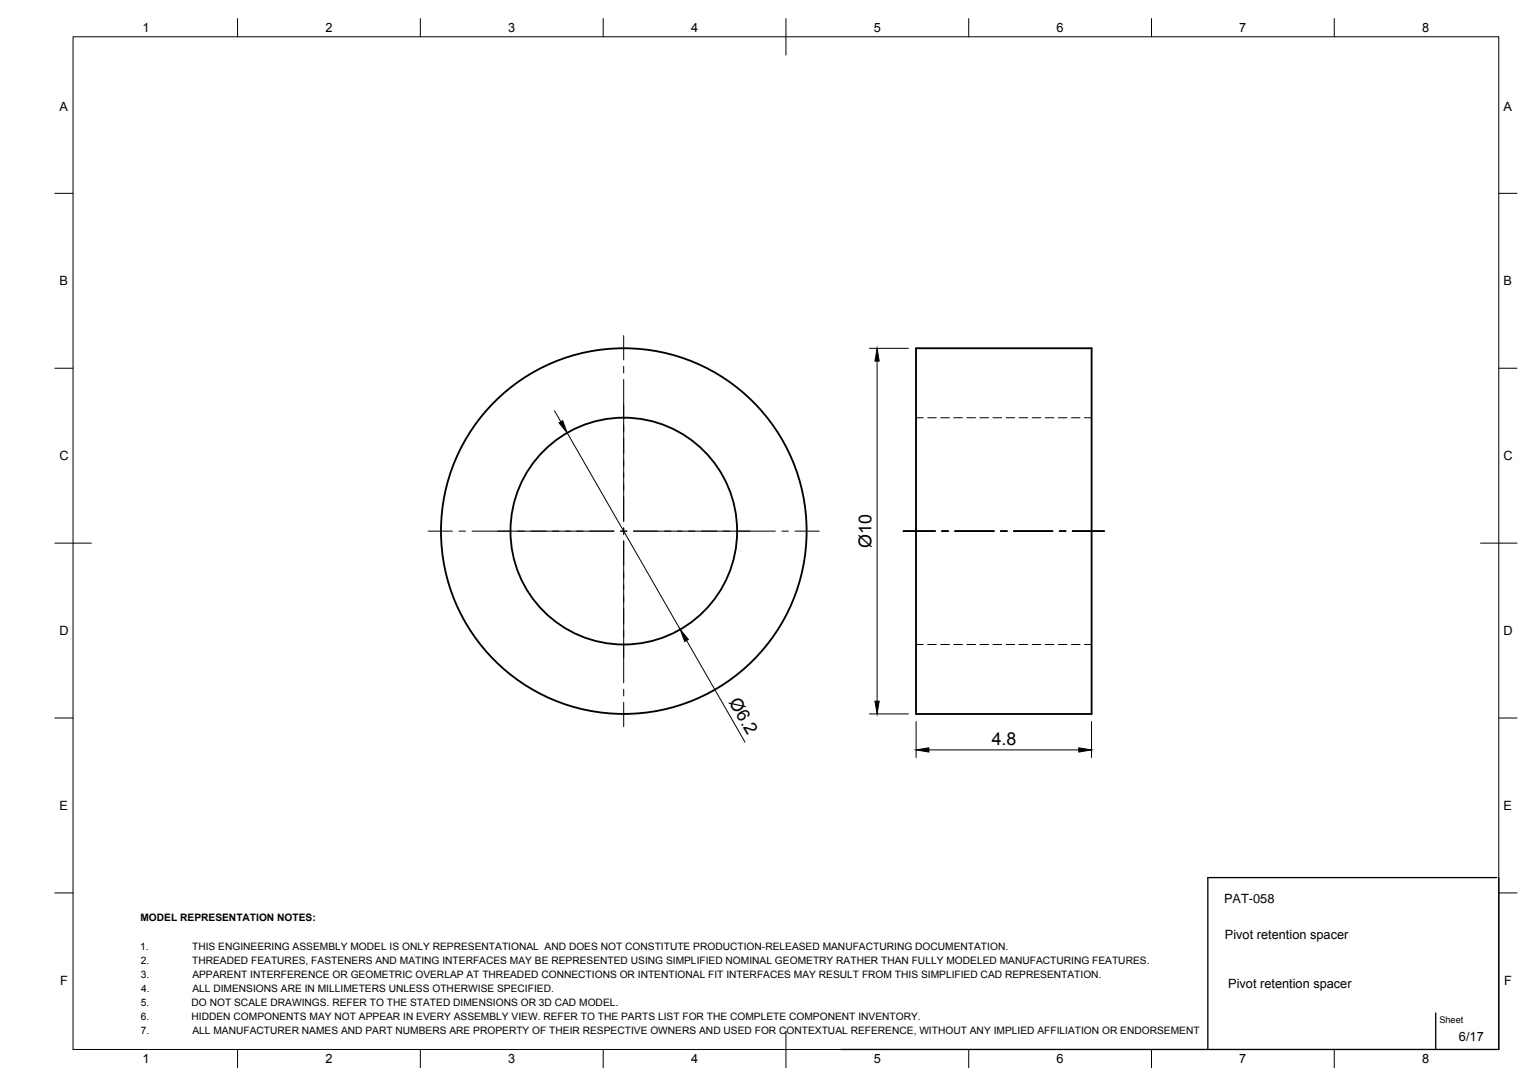
ISO-10303-21;
HEADER;
/* Generated by software containing ST-Developer
 * from STEP Tools, Inc. (www.steptools.com) 
 */

FILE_DESCRIPTION(
/* description */ ('Horizontal push-pull toggle clamp'),
/* implementation_level */ '2;1');

FILE_NAME(
/* name */ 'Pivot retention spacer.step',
/* time_stamp */ '2026-10-27T21:21:09-07:00',
/* author */ (''),
/* organization */ (''),
/* preprocessor_version */ 'ST-DEVELOPER v20.2',
/* originating_system */ 'Autodesk Translation Framework v15.17.0.0',
/* authorisation */ '');

FILE_SCHEMA (('AUTOMOTIVE_DESIGN { 1 0 10303 214 3 1 1 }'));
ENDSEC;

DATA;
#10=MECHANICAL_DESIGN_GEOMETRIC_PRESENTATION_REPRESENTATION('',(#196),#4791);
#170=SHAPE_REPRESENTATION_RELATIONSHIP('SRR','None',#4876,#183);
#183=ADVANCED_BREP_SHAPE_REPRESENTATION('',(#208),#4789);
#196=STYLED_ITEM('',(#5037),#208);
#208=MANIFOLD_SOLID_BREP('Body1',#2641);
#253=FACE_BOUND('',#701,.T.);
#254=FACE_BOUND('',#703,.T.);
#357=PLANE('',#3030);
#358=PLANE('',#3031);
#504=FACE_OUTER_BOUND('',#698,.T.);
#505=FACE_OUTER_BOUND('',#699,.T.);
#506=FACE_OUTER_BOUND('',#700,.T.);
#507=FACE_OUTER_BOUND('',#702,.T.);
#698=EDGE_LOOP('',(#2407,#2408,#2409,#2410));
#699=EDGE_LOOP('',(#2411,#2412,#2413,#2414));
#700=EDGE_LOOP('',(#2415));
#701=EDGE_LOOP('',(#2416));
#702=EDGE_LOOP('',(#2417));
#703=EDGE_LOOP('',(#2418));
#787=CIRCLE('',#3025,0.31);
#788=CIRCLE('',#3026,0.31);
#789=CIRCLE('',#3028,0.5);
#790=CIRCLE('',#3029,0.5);
#1009=LINE('',#4641,#1229);
#1010=LINE('',#4647,#1230);
#1229=VECTOR('',#3761,0.31);
#1230=VECTOR('',#3768,0.5);
#1441=VERTEX_POINT('',#4638);
#1442=VERTEX_POINT('',#4640);
#1443=VERTEX_POINT('',#4644);
#1444=VERTEX_POINT('',#4646);
#1765=EDGE_CURVE('',#1441,#1441,#787,.T.);
#1766=EDGE_CURVE('',#1441,#1442,#1009,.T.);
#1767=EDGE_CURVE('',#1442,#1442,#788,.T.);
#1768=EDGE_CURVE('',#1443,#1443,#789,.T.);
#1769=EDGE_CURVE('',#1443,#1444,#1010,.T.);
#1770=EDGE_CURVE('',#1444,#1444,#790,.T.);
#2407=ORIENTED_EDGE('',*,*,#1765,.F.);
#2408=ORIENTED_EDGE('',*,*,#1766,.T.);
#2409=ORIENTED_EDGE('',*,*,#1767,.T.);
#2410=ORIENTED_EDGE('',*,*,#1766,.F.);
#2411=ORIENTED_EDGE('',*,*,#1768,.F.);
#2412=ORIENTED_EDGE('',*,*,#1769,.T.);
#2413=ORIENTED_EDGE('',*,*,#1770,.T.);
#2414=ORIENTED_EDGE('',*,*,#1769,.F.);
#2415=ORIENTED_EDGE('',*,*,#1768,.T.);
#2416=ORIENTED_EDGE('',*,*,#1765,.T.);
#2417=ORIENTED_EDGE('',*,*,#1770,.F.);
#2418=ORIENTED_EDGE('',*,*,#1767,.F.);
#2475=CYLINDRICAL_SURFACE('',#3024,0.31);
#2476=CYLINDRICAL_SURFACE('',#3027,0.5);
#2620=ADVANCED_FACE('',(#504),#2475,.F.);
#2621=ADVANCED_FACE('',(#505),#2476,.T.);
#2622=ADVANCED_FACE('',(#506,#253),#357,.T.);
#2623=ADVANCED_FACE('',(#507,#254),#358,.F.);
#2641=CLOSED_SHELL('',(#2620,#2621,#2622,#2623));
#3023=AXIS2_PLACEMENT_3D('',#4636,#3755,#3756);
#3024=AXIS2_PLACEMENT_3D('',#4637,#3757,#3758);
#3025=AXIS2_PLACEMENT_3D('',#4639,#3759,#3760);
#3026=AXIS2_PLACEMENT_3D('',#4642,#3762,#3763);
#3027=AXIS2_PLACEMENT_3D('',#4643,#3764,#3765);
#3028=AXIS2_PLACEMENT_3D('',#4645,#3766,#3767);
#3029=AXIS2_PLACEMENT_3D('',#4648,#3769,#3770);
#3030=AXIS2_PLACEMENT_3D('',#4649,#3771,#3772);
#3031=AXIS2_PLACEMENT_3D('',#4650,#3773,#3774);
#3755=DIRECTION('axis',(0.,0.,1.));
#3756=DIRECTION('refdir',(1.,0.,0.));
#3757=DIRECTION('center_axis',(0.,1.,0.));
#3758=DIRECTION('ref_axis',(1.,0.,0.));
#3759=DIRECTION('center_axis',(0.,-1.,0.));
#3760=DIRECTION('ref_axis',(1.,0.,0.));
#3761=DIRECTION('',(0.,-1.,0.));
#3762=DIRECTION('center_axis',(0.,-1.,0.));
#3763=DIRECTION('ref_axis',(1.,0.,0.));
#3764=DIRECTION('center_axis',(0.,1.,0.));
#3765=DIRECTION('ref_axis',(1.,0.,0.));
#3766=DIRECTION('center_axis',(0.,1.,0.));
#3767=DIRECTION('ref_axis',(1.,0.,0.));
#3768=DIRECTION('',(0.,-1.,0.));
#3769=DIRECTION('center_axis',(0.,1.,0.));
#3770=DIRECTION('ref_axis',(1.,0.,0.));
#3771=DIRECTION('center_axis',(0.,1.,0.));
#3772=DIRECTION('ref_axis',(1.,0.,0.));
#3773=DIRECTION('center_axis',(0.,1.,0.));
#3774=DIRECTION('ref_axis',(1.,0.,0.));
#4636=CARTESIAN_POINT('',(0.,0.,0.));
#4637=CARTESIAN_POINT('Origin',(0.,-1.54,2.5));
#4638=CARTESIAN_POINT('',(-0.31,-1.06,2.5));
#4639=CARTESIAN_POINT('Origin',(0.,-1.06,2.5));
#4640=CARTESIAN_POINT('',(-0.31,-1.54,2.5));
#4641=CARTESIAN_POINT('',(-0.31,-1.54,2.5));
#4642=CARTESIAN_POINT('Origin',(0.,-1.54,2.5));
#4643=CARTESIAN_POINT('Origin',(0.,-1.54,2.5));
#4644=CARTESIAN_POINT('',(-0.5,-1.06,2.5));
#4645=CARTESIAN_POINT('Origin',(0.,-1.06,2.5));
#4646=CARTESIAN_POINT('',(-0.5,-1.54,2.5));
#4647=CARTESIAN_POINT('',(-0.5,-1.54,2.5));
#4648=CARTESIAN_POINT('Origin',(0.,-1.54,2.5));
#4649=CARTESIAN_POINT('Origin',(0.,-1.06,2.5));
#4650=CARTESIAN_POINT('Origin',(0.,-1.54,2.5));
#4770=UNCERTAINTY_MEASURE_WITH_UNIT(LENGTH_MEASURE(0.001),#4792,
'DISTANCE_ACCURACY_VALUE',
'Maximum model space distance between geometric entities at asserted c
onnectivities');
#4772=UNCERTAINTY_MEASURE_WITH_UNIT(LENGTH_MEASURE(0.001),#4792,
'DISTANCE_ACCURACY_VALUE',
'Maximum model space distance between geometric entities at asserted c
onnectivities');
#4789=(
GEOMETRIC_REPRESENTATION_CONTEXT(3)
GLOBAL_UNCERTAINTY_ASSIGNED_CONTEXT((#4770))
GLOBAL_UNIT_ASSIGNED_CONTEXT((#4792,#4794,#4795))
REPRESENTATION_CONTEXT('','3D')
);
#4791=(
GEOMETRIC_REPRESENTATION_CONTEXT(3)
GLOBAL_UNCERTAINTY_ASSIGNED_CONTEXT((#4772))
GLOBAL_UNIT_ASSIGNED_CONTEXT((#4792,#4794,#4795))
REPRESENTATION_CONTEXT('','3D')
);
#4792=(
LENGTH_UNIT()
NAMED_UNIT(*)
SI_UNIT(.CENTI.,.METRE.)
);
#4794=(
NAMED_UNIT(*)
PLANE_ANGLE_UNIT()
SI_UNIT($,.RADIAN.)
);
#4795=(
NAMED_UNIT(*)
SI_UNIT($,.STERADIAN.)
SOLID_ANGLE_UNIT()
);
#4812=SHAPE_DEFINITION_REPRESENTATION(#4831,#4876);
#4831=PRODUCT_DEFINITION_SHAPE('',$,#4895);
#4876=SHAPE_REPRESENTATION('',(#3023),#4789);
#4878=PRODUCT_DEFINITION_CONTEXT('part definition',#4934,'design');
#4895=PRODUCT_DEFINITION('Pivot retention spacer',
'Pivot retention spacer',#4913,#4878);
#4913=PRODUCT_DEFINITION_FORMATION('',$,#4952);
#4934=APPLICATION_CONTEXT(
'Core Data for Automotive Mechanical Design Process');
#4935=PRODUCT_CONTEXT('part definition',#4934,'mechanical');
#4952=PRODUCT('Pivot retention spacer','Pivot retention spacer',
'Pivot retention spacer',(#4935));
#5031=COLOUR_RGB('Off White',0.89,0.88,0.83);
#5032=FILL_AREA_STYLE_COLOUR('',#5031);
#5033=FILL_AREA_STYLE('',(#5032));
#5034=SURFACE_STYLE_FILL_AREA(#5033);
#5035=SURFACE_SIDE_STYLE('',(#5034));
#5036=SURFACE_STYLE_USAGE(.BOTH.,#5035);
#5037=PRESENTATION_STYLE_ASSIGNMENT((#5036));
ENDSEC;
END-ISO-10303-21;
